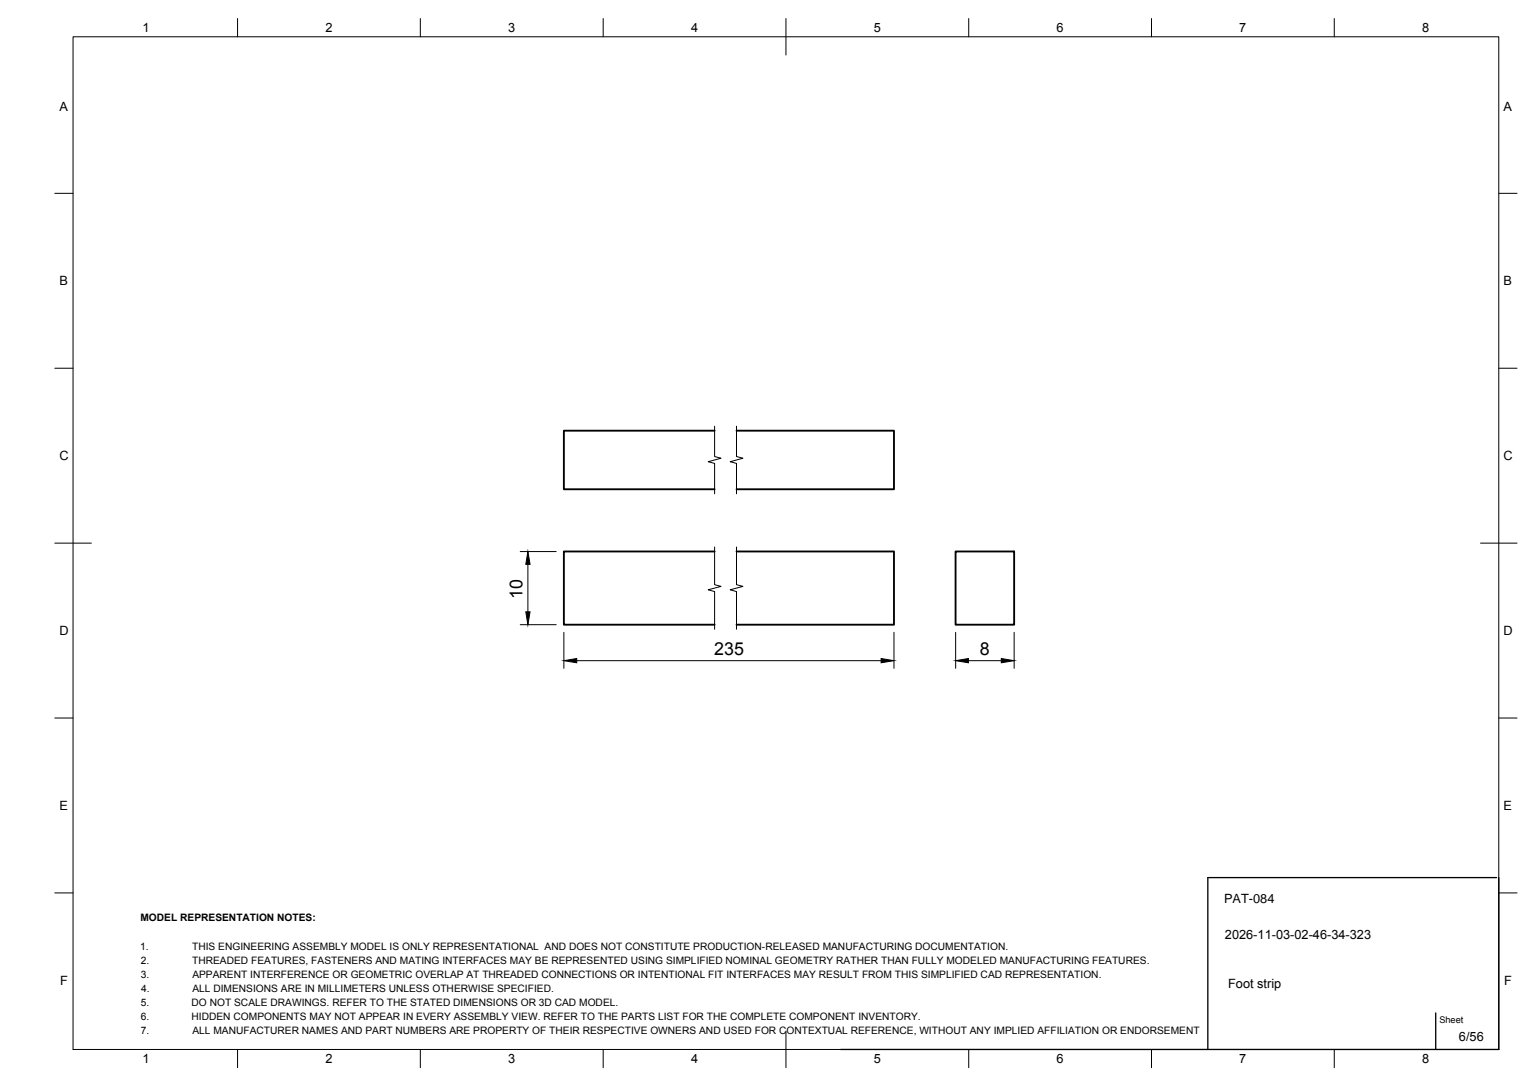
ISO-10303-21;
HEADER;
/* Generated by software containing ST-Developer
 * from STEP Tools, Inc. (www.steptools.com) 
 */

FILE_DESCRIPTION(
/* description */ ('Quick-return (Whitworth) mechanism'),
/* implementation_level */ '2;1');

FILE_NAME(
/* name */ 'Foot strip.step',
/* time_stamp */ '2026-10-28T03:25:57-07:00',
/* author */ (''),
/* organization */ (''),
/* preprocessor_version */ 'ST-DEVELOPER v20.2',
/* originating_system */ 'Autodesk Translation Framework v15.17.0.0',
/* authorisation */ '');

FILE_SCHEMA (('AUTOMOTIVE_DESIGN { 1 0 10303 214 3 1 1 }'));
ENDSEC;

DATA;
#10=MECHANICAL_DESIGN_GEOMETRIC_PRESENTATION_REPRESENTATION('',(#491),#14878);
#403=SHAPE_REPRESENTATION_RELATIONSHIP('SRR','None',#15071,#447);
#447=ADVANCED_BREP_SHAPE_REPRESENTATION('',(#543),#14828);
#491=STYLED_ITEM('',(#15392),#543);
#543=MANIFOLD_SOLID_BREP('Body1',#7845);
#788=PLANE('',#8430);
#789=PLANE('',#8431);
#790=PLANE('',#8432);
#791=PLANE('',#8433);
#792=PLANE('',#8434);
#793=PLANE('',#8435);
#1065=FACE_OUTER_BOUND('',#1555,.T.);
#1066=FACE_OUTER_BOUND('',#1556,.T.);
#1067=FACE_OUTER_BOUND('',#1557,.T.);
#1068=FACE_OUTER_BOUND('',#1558,.T.);
#1069=FACE_OUTER_BOUND('',#1559,.T.);
#1070=FACE_OUTER_BOUND('',#1560,.T.);
#1555=EDGE_LOOP('',(#5358,#5359,#5360,#5361));
#1556=EDGE_LOOP('',(#5362,#5363,#5364,#5365));
#1557=EDGE_LOOP('',(#5366,#5367,#5368,#5369));
#1558=EDGE_LOOP('',(#5370,#5371,#5372,#5373));
#1559=EDGE_LOOP('',(#5374,#5375,#5376,#5377));
#1560=EDGE_LOOP('',(#5378,#5379,#5380,#5381));
#2194=LINE('',#12051,#2717);
#2195=LINE('',#12053,#2718);
#2196=LINE('',#12055,#2719);
#2197=LINE('',#12056,#2720);
#2198=LINE('',#12059,#2721);
#2199=LINE('',#12061,#2722);
#2200=LINE('',#12062,#2723);
#2201=LINE('',#12065,#2724);
#2202=LINE('',#12067,#2725);
#2203=LINE('',#12068,#2726);
#2204=LINE('',#12070,#2727);
#2205=LINE('',#12071,#2728);
#2717=VECTOR('',#9515,1.);
#2718=VECTOR('',#9516,1.);
#2719=VECTOR('',#9517,1.);
#2720=VECTOR('',#9518,1.);
#2721=VECTOR('',#9521,1.);
#2722=VECTOR('',#9522,1.);
#2723=VECTOR('',#9523,1.);
#2724=VECTOR('',#9526,1.);
#2725=VECTOR('',#9527,1.);
#2726=VECTOR('',#9528,1.);
#2727=VECTOR('',#9531,1.);
#2728=VECTOR('',#9532,1.);
#3663=VERTEX_POINT('',#12049);
#3664=VERTEX_POINT('',#12050);
#3665=VERTEX_POINT('',#12052);
#3666=VERTEX_POINT('',#12054);
#3667=VERTEX_POINT('',#12058);
#3668=VERTEX_POINT('',#12060);
#3669=VERTEX_POINT('',#12064);
#3670=VERTEX_POINT('',#12066);
#4336=EDGE_CURVE('',#3663,#3664,#2194,.T.);
#4337=EDGE_CURVE('',#3664,#3665,#2195,.T.);
#4338=EDGE_CURVE('',#3666,#3665,#2196,.T.);
#4339=EDGE_CURVE('',#3663,#3666,#2197,.T.);
#4340=EDGE_CURVE('',#3667,#3663,#2198,.T.);
#4341=EDGE_CURVE('',#3668,#3666,#2199,.T.);
#4342=EDGE_CURVE('',#3667,#3668,#2200,.T.);
#4343=EDGE_CURVE('',#3669,#3667,#2201,.T.);
#4344=EDGE_CURVE('',#3670,#3668,#2202,.T.);
#4345=EDGE_CURVE('',#3669,#3670,#2203,.T.);
#4346=EDGE_CURVE('',#3664,#3669,#2204,.T.);
#4347=EDGE_CURVE('',#3665,#3670,#2205,.T.);
#5358=ORIENTED_EDGE('',*,*,#4336,.T.);
#5359=ORIENTED_EDGE('',*,*,#4337,.T.);
#5360=ORIENTED_EDGE('',*,*,#4338,.F.);
#5361=ORIENTED_EDGE('',*,*,#4339,.F.);
#5362=ORIENTED_EDGE('',*,*,#4340,.T.);
#5363=ORIENTED_EDGE('',*,*,#4339,.T.);
#5364=ORIENTED_EDGE('',*,*,#4341,.F.);
#5365=ORIENTED_EDGE('',*,*,#4342,.F.);
#5366=ORIENTED_EDGE('',*,*,#4343,.T.);
#5367=ORIENTED_EDGE('',*,*,#4342,.T.);
#5368=ORIENTED_EDGE('',*,*,#4344,.F.);
#5369=ORIENTED_EDGE('',*,*,#4345,.F.);
#5370=ORIENTED_EDGE('',*,*,#4346,.T.);
#5371=ORIENTED_EDGE('',*,*,#4345,.T.);
#5372=ORIENTED_EDGE('',*,*,#4347,.F.);
#5373=ORIENTED_EDGE('',*,*,#4337,.F.);
#5374=ORIENTED_EDGE('',*,*,#4347,.T.);
#5375=ORIENTED_EDGE('',*,*,#4344,.T.);
#5376=ORIENTED_EDGE('',*,*,#4341,.T.);
#5377=ORIENTED_EDGE('',*,*,#4338,.T.);
#5378=ORIENTED_EDGE('',*,*,#4346,.F.);
#5379=ORIENTED_EDGE('',*,*,#4336,.F.);
#5380=ORIENTED_EDGE('',*,*,#4340,.F.);
#5381=ORIENTED_EDGE('',*,*,#4343,.F.);
#7396=ADVANCED_FACE('',(#1065),#788,.T.);
#7397=ADVANCED_FACE('',(#1066),#789,.T.);
#7398=ADVANCED_FACE('',(#1067),#790,.T.);
#7399=ADVANCED_FACE('',(#1068),#791,.T.);
#7400=ADVANCED_FACE('',(#1069),#792,.T.);
#7401=ADVANCED_FACE('',(#1070),#793,.F.);
#7845=CLOSED_SHELL('',(#7396,#7397,#7398,#7399,#7400,#7401));
#8429=AXIS2_PLACEMENT_3D('',#12047,#9511,#9512);
#8430=AXIS2_PLACEMENT_3D('',#12048,#9513,#9514);
#8431=AXIS2_PLACEMENT_3D('',#12057,#9519,#9520);
#8432=AXIS2_PLACEMENT_3D('',#12063,#9524,#9525);
#8433=AXIS2_PLACEMENT_3D('',#12069,#9529,#9530);
#8434=AXIS2_PLACEMENT_3D('',#12072,#9533,#9534);
#8435=AXIS2_PLACEMENT_3D('',#12073,#9535,#9536);
#9511=DIRECTION('axis',(0.,0.,1.));
#9512=DIRECTION('refdir',(1.,0.,0.));
#9513=DIRECTION('center_axis',(0.,1.,0.));
#9514=DIRECTION('ref_axis',(-1.,0.,0.));
#9515=DIRECTION('',(-1.,0.,0.));
#9516=DIRECTION('',(0.,0.,1.));
#9517=DIRECTION('',(-1.,0.,0.));
#9518=DIRECTION('',(0.,0.,1.));
#9519=DIRECTION('center_axis',(1.,0.,0.));
#9520=DIRECTION('ref_axis',(0.,1.,0.));
#9521=DIRECTION('',(0.,1.,0.));
#9522=DIRECTION('',(0.,1.,0.));
#9523=DIRECTION('',(0.,0.,1.));
#9524=DIRECTION('center_axis',(0.,-1.,0.));
#9525=DIRECTION('ref_axis',(1.,0.,0.));
#9526=DIRECTION('',(1.,0.,0.));
#9527=DIRECTION('',(1.,0.,0.));
#9528=DIRECTION('',(0.,0.,1.));
#9529=DIRECTION('center_axis',(-1.,0.,0.));
#9530=DIRECTION('ref_axis',(0.,-1.,0.));
#9531=DIRECTION('',(0.,-1.,0.));
#9532=DIRECTION('',(0.,-1.,0.));
#9533=DIRECTION('center_axis',(0.,0.,1.));
#9534=DIRECTION('ref_axis',(1.,0.,0.));
#9535=DIRECTION('center_axis',(0.,0.,1.));
#9536=DIRECTION('ref_axis',(1.,0.,0.));
#12047=CARTESIAN_POINT('',(0.,0.,0.));
#12048=CARTESIAN_POINT('Origin',(-8.,20.,-0.8));
#12049=CARTESIAN_POINT('',(-8.,20.,-0.8));
#12050=CARTESIAN_POINT('',(-9.,20.,-0.8));
#12051=CARTESIAN_POINT('',(-8.,20.,-0.8));
#12052=CARTESIAN_POINT('',(-9.,20.,0.));
#12053=CARTESIAN_POINT('',(-9.,20.,-0.8));
#12054=CARTESIAN_POINT('',(-8.,20.,0.));
#12055=CARTESIAN_POINT('',(-8.,20.,0.));
#12056=CARTESIAN_POINT('',(-8.,20.,-0.8));
#12057=CARTESIAN_POINT('Origin',(-8.,-3.5,-0.8));
#12058=CARTESIAN_POINT('',(-8.,-3.5,-0.8));
#12059=CARTESIAN_POINT('',(-8.,-3.5,-0.8));
#12060=CARTESIAN_POINT('',(-8.,-3.5,0.));
#12061=CARTESIAN_POINT('',(-8.,-3.5,0.));
#12062=CARTESIAN_POINT('',(-8.,-3.5,-0.8));
#12063=CARTESIAN_POINT('Origin',(-9.,-3.5,-0.8));
#12064=CARTESIAN_POINT('',(-9.,-3.5,-0.8));
#12065=CARTESIAN_POINT('',(-9.,-3.5,-0.8));
#12066=CARTESIAN_POINT('',(-9.,-3.5,0.));
#12067=CARTESIAN_POINT('',(-9.,-3.5,0.));
#12068=CARTESIAN_POINT('',(-9.,-3.5,-0.8));
#12069=CARTESIAN_POINT('Origin',(-9.,20.,-0.8));
#12070=CARTESIAN_POINT('',(-9.,20.,-0.8));
#12071=CARTESIAN_POINT('',(-9.,20.,0.));
#12072=CARTESIAN_POINT('Origin',(-8.5,8.25,0.));
#12073=CARTESIAN_POINT('Origin',(-8.5,8.25,-0.8));
#14774=UNCERTAINTY_MEASURE_WITH_UNIT(LENGTH_MEASURE(0.001),#14879,
'DISTANCE_ACCURACY_VALUE',
'Maximum model space distance between geometric entities at asserted c
onnectivities');
#14824=UNCERTAINTY_MEASURE_WITH_UNIT(LENGTH_MEASURE(0.001),#14879,
'DISTANCE_ACCURACY_VALUE',
'Maximum model space distance between geometric entities at asserted c
onnectivities');
#14828=(
GEOMETRIC_REPRESENTATION_CONTEXT(3)
GLOBAL_UNCERTAINTY_ASSIGNED_CONTEXT((#14774))
GLOBAL_UNIT_ASSIGNED_CONTEXT((#14879,#14881,#14882))
REPRESENTATION_CONTEXT('','3D')
);
#14878=(
GEOMETRIC_REPRESENTATION_CONTEXT(3)
GLOBAL_UNCERTAINTY_ASSIGNED_CONTEXT((#14824))
GLOBAL_UNIT_ASSIGNED_CONTEXT((#14879,#14881,#14882))
REPRESENTATION_CONTEXT('','3D')
);
#14879=(
LENGTH_UNIT()
NAMED_UNIT(*)
SI_UNIT(.CENTI.,.METRE.)
);
#14881=(
NAMED_UNIT(*)
PLANE_ANGLE_UNIT()
SI_UNIT($,.RADIAN.)
);
#14882=(
NAMED_UNIT(*)
SI_UNIT($,.STERADIAN.)
SOLID_ANGLE_UNIT()
);
#14886=SHAPE_DEFINITION_REPRESENTATION(#14939,#15071);
#14939=PRODUCT_DEFINITION_SHAPE('',$,#15125);
#15071=SHAPE_REPRESENTATION('',(#8429),#14828);
#15121=PRODUCT_DEFINITION_CONTEXT('part definition',#15282,'design');
#15125=PRODUCT_DEFINITION('Foot strip','Foot strip',#15178,#15121);
#15178=PRODUCT_DEFINITION_FORMATION('',$,#15287);
#15282=APPLICATION_CONTEXT(
'Core Data for Automotive Mechanical Design Process');
#15283=PRODUCT_CONTEXT('part definition',#15282,'mechanical');
#15287=PRODUCT('Foot strip','Foot strip','Foot strip',(#15283));
#15386=COLOUR_RGB('Light Blue',0.38,0.62,0.78);
#15387=FILL_AREA_STYLE_COLOUR('',#15386);
#15388=FILL_AREA_STYLE('',(#15387));
#15389=SURFACE_STYLE_FILL_AREA(#15388);
#15390=SURFACE_SIDE_STYLE('',(#15389));
#15391=SURFACE_STYLE_USAGE(.BOTH.,#15390);
#15392=PRESENTATION_STYLE_ASSIGNMENT((#15391));
ENDSEC;
END-ISO-10303-21;
